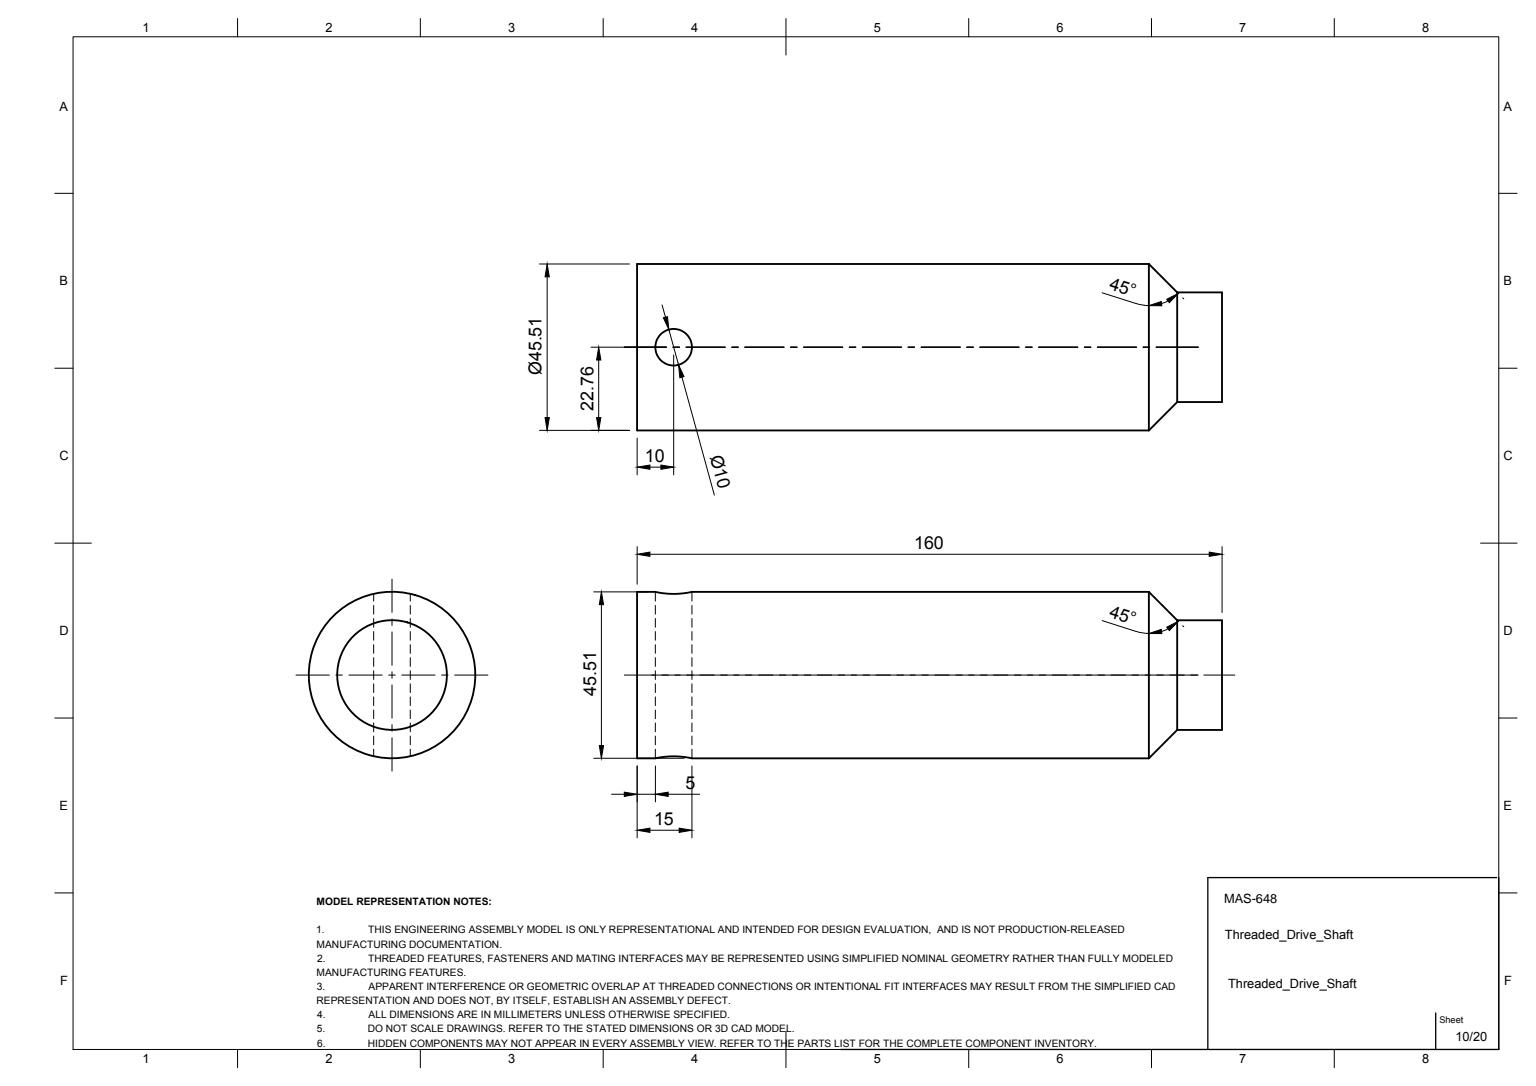
ISO-10303-21;
HEADER;
FILE_DESCRIPTION((''),'2;1');
FILE_NAME('Threaded_Drive_Shaft.step','2026-10-09T12:47:58-07:00',(''),(''),'','','');
FILE_SCHEMA (('AUTOMOTIVE_DESIGN { 1 0 10303 214 3 1 1 }'));
ENDSEC;
DATA;
#10=MECHANICAL_DESIGN_GEOMETRIC_PRESENTATION_REPRESENTATION('',(#313),#3475);
#31=CONICAL_SURFACE('',#2014,22.7551020408163,0.785398163397443) ;
#41=B_SPLINE_CURVE_WITH_KNOTS('',3,(#2969,#2970,#2971,#2972,#2973,#2974,
#2975,#2976,#2977,#2978,#2979,#2980,#2981,#2982,#2983,#2984,#2985,#2986,
#2987),.UNSPECIFIED.,.F.,.F.,(4,2,2,2,3,2,2,2,4),(-0.756034971359867,-0.567034005964369,
-0.378033040568871,-0.189016520284436,0.,0.189016520284436,0.378033040568871,
0.567034005964369,0.756034971359867),.UNSPECIFIED.) ;
#42=B_SPLINE_CURVE_WITH_KNOTS('',3,(#2989,#2990,#2991,#2992,#2993,#2994,
#2995,#2996,#2997,#2998),.UNSPECIFIED.,.F.,.F.,(4,2,2,2,4),(0.756034971359867,
0.945035936755365,1.13403690215086,1.3230534224353,1.51206994271973),
 .UNSPECIFIED.) ;
#43=B_SPLINE_CURVE_WITH_KNOTS('',3,(#3001,#3002,#3003,#3004,#3005,#3006,
#3007,#3008,#3009,#3010,#3011,#3012,#3013,#3014,#3015,#3016,#3017,#3018,
#3019,#3020,#3021,#3022,#3023,#3024,#3025,#3026,#3027,#3028,#3029,#3030,
#3031,#3032,#3033,#3034),.UNSPECIFIED.,.T.,.F.,(4,2,2,2,2,2,2,2,2,2,2,2,
2,2,2,2,4),(-3.02413988543947,-2.83512336515503,-2.6461068448706,-2.4571058794751,
-2.2681049140796,-2.0791039486841,-1.8901029832886,-1.70108646300417,-1.51206994271973,
-1.3230534224353,-1.13403690215086,-0.945035936755364,-0.756034971359867,
-0.567034005964369,-0.378033040568871,-0.189016520284436,0.),
 .UNSPECIFIED.) ;
#44=B_SPLINE_CURVE_WITH_KNOTS('',3,(#3035,#3036,#3037,#3038,#3039,#3040,
#3041,#3042,#3043,#3044),.UNSPECIFIED.,.F.,.F.,(4,2,2,2,4),(1.51206994271973,
1.70108646300417,1.8901029832886,2.0791039486841,2.2681049140796),
 .UNSPECIFIED.) ;
#147=FACE_BOUND('',#484,.T.) ;
#172=CIRCLE('',#2015,22.7551020408163) ;
#173=CIRCLE('',#2016,15.) ;
#174=CIRCLE('',#2018,22.7551020408163) ;
#175=CIRCLE('',#2020,15.) ;
#259=CYLINDRICAL_SURFACE('',#2013,5.00000000000002) ;
#260=CYLINDRICAL_SURFACE('',#2017,22.7551020408163) ;
#261=CYLINDRICAL_SURFACE('',#2019,15.) ;
#289=SHAPE_REPRESENTATION_RELATIONSHIP('SRR','None',#3544,#301) ;
#301=ADVANCED_BREP_SHAPE_REPRESENTATION('',(#325),#3464) ;
#313=STYLED_ITEM('',(#3628),#325) ;
#325=MANIFOLD_SOLID_BREP('Body1',#1827) ;
#361=FACE_OUTER_BOUND('',#481,.T.) ;
#362=FACE_OUTER_BOUND('',#482,.T.) ;
#363=FACE_OUTER_BOUND('',#483,.T.) ;
#364=FACE_OUTER_BOUND('',#485,.T.) ;
#365=FACE_OUTER_BOUND('',#486,.T.) ;
#366=FACE_OUTER_BOUND('',#487,.T.) ;
#481=EDGE_LOOP('',(#1320,#1321,#1322,#1323,#1324,#1325)) ;
#482=EDGE_LOOP('',(#1326,#1327,#1328,#1329)) ;
#483=EDGE_LOOP('',(#1330,#1331,#1332,#1333,#1334,#1335,#1336,#1337,#1338)) ;
#484=EDGE_LOOP('',(#1339)) ;
#485=EDGE_LOOP('',(#1340,#1341,#1342,#1343)) ;
#486=EDGE_LOOP('',(#1344)) ;
#487=EDGE_LOOP('',(#1345)) ;
#644=LINE('',#3000,#763) ;
#645=LINE('',#3049,#764) ;
#646=LINE('',#3054,#765) ;
#647=LINE('',#3055,#766) ;
#648=LINE('',#3058,#767) ;
#763=VECTOR('',#2361,5.00000000000002) ;
#764=VECTOR('',#2366,22.7551020408163) ;
#765=VECTOR('',#2373,22.7551020408163) ;
#766=VECTOR('',#2374,22.7551020408163) ;
#767=VECTOR('',#2377,15.) ;
#867=VERTEX_POINT('',#2967) ;
#868=VERTEX_POINT('',#2968) ;
#869=VERTEX_POINT('',#2988) ;
#870=VERTEX_POINT('',#2999) ;
#871=VERTEX_POINT('',#3046) ;
#872=VERTEX_POINT('',#3048) ;
#873=VERTEX_POINT('',#3052) ;
#874=VERTEX_POINT('',#3057) ;
#1032=EDGE_CURVE('',#867,#868,#41,.T.) ;
#1033=EDGE_CURVE('',#868,#869,#42,.T.) ;
#1034=EDGE_CURVE('',#869,#870,#644,.T.) ;
#1035=EDGE_CURVE('',#870,#870,#43,.T.) ;
#1036=EDGE_CURVE('',#869,#867,#44,.T.) ;
#1037=EDGE_CURVE('',#871,#871,#172,.T.) ;
#1038=EDGE_CURVE('',#871,#872,#645,.T.) ;
#1039=EDGE_CURVE('',#872,#872,#173,.T.) ;
#1040=EDGE_CURVE('',#873,#873,#174,.T.) ;
#1041=EDGE_CURVE('',#873,#867,#646,.T.) ;
#1042=EDGE_CURVE('',#868,#871,#647,.T.) ;
#1043=EDGE_CURVE('',#872,#874,#648,.T.) ;
#1044=EDGE_CURVE('',#874,#874,#175,.T.) ;
#1320=ORIENTED_EDGE('',*,*,#1032,.T.) ;
#1321=ORIENTED_EDGE('',*,*,#1033,.T.) ;
#1322=ORIENTED_EDGE('',*,*,#1034,.T.) ;
#1323=ORIENTED_EDGE('',*,*,#1035,.T.) ;
#1324=ORIENTED_EDGE('',*,*,#1034,.F.) ;
#1325=ORIENTED_EDGE('',*,*,#1036,.T.) ;
#1326=ORIENTED_EDGE('',*,*,#1037,.F.) ;
#1327=ORIENTED_EDGE('',*,*,#1038,.T.) ;
#1328=ORIENTED_EDGE('',*,*,#1039,.F.) ;
#1329=ORIENTED_EDGE('',*,*,#1038,.F.) ;
#1330=ORIENTED_EDGE('',*,*,#1040,.F.) ;
#1331=ORIENTED_EDGE('',*,*,#1041,.T.) ;
#1332=ORIENTED_EDGE('',*,*,#1036,.F.) ;
#1333=ORIENTED_EDGE('',*,*,#1033,.F.) ;
#1334=ORIENTED_EDGE('',*,*,#1042,.T.) ;
#1335=ORIENTED_EDGE('',*,*,#1037,.T.) ;
#1336=ORIENTED_EDGE('',*,*,#1042,.F.) ;
#1337=ORIENTED_EDGE('',*,*,#1032,.F.) ;
#1338=ORIENTED_EDGE('',*,*,#1041,.F.) ;
#1339=ORIENTED_EDGE('',*,*,#1035,.F.) ;
#1340=ORIENTED_EDGE('',*,*,#1039,.T.) ;
#1341=ORIENTED_EDGE('',*,*,#1043,.T.) ;
#1342=ORIENTED_EDGE('',*,*,#1044,.T.) ;
#1343=ORIENTED_EDGE('',*,*,#1043,.F.) ;
#1344=ORIENTED_EDGE('',*,*,#1044,.F.) ;
#1345=ORIENTED_EDGE('',*,*,#1040,.T.) ;
#1668=PLANE('',#2021) ;
#1669=PLANE('',#2022) ;
#1737=ADVANCED_FACE('',(#361),#259,.F.) ;
#1738=ADVANCED_FACE('',(#362),#31,.T.) ;
#1739=ADVANCED_FACE('',(#363,#147),#260,.T.) ;
#1740=ADVANCED_FACE('',(#364),#261,.T.) ;
#1741=ADVANCED_FACE('',(#365),#1668,.T.) ;
#1742=ADVANCED_FACE('',(#366),#1669,.T.) ;
#1827=CLOSED_SHELL('',(#1737,#1738,#1739,#1740,#1741,#1742)) ;
#2012=AXIS2_PLACEMENT_3D('',#2965,#2357,#2358) ;
#2013=AXIS2_PLACEMENT_3D('',#2966,#2359,#2360) ;
#2014=AXIS2_PLACEMENT_3D('',#3045,#2362,#2363) ;
#2015=AXIS2_PLACEMENT_3D('',#3047,#2364,#2365) ;
#2016=AXIS2_PLACEMENT_3D('',#3050,#2367,#2368) ;
#2017=AXIS2_PLACEMENT_3D('',#3051,#2369,#2370) ;
#2018=AXIS2_PLACEMENT_3D('',#3053,#2371,#2372) ;
#2019=AXIS2_PLACEMENT_3D('',#3056,#2375,#2376) ;
#2020=AXIS2_PLACEMENT_3D('',#3059,#2378,#2379) ;
#2021=AXIS2_PLACEMENT_3D('',#3060,#2380,#2381) ;
#2022=AXIS2_PLACEMENT_3D('',#3061,#2382,#2383) ;
#2357=DIRECTION('axis',(0.,0.,1.)) ;
#2358=DIRECTION('refdir',(1.,0.,0.)) ;
#2359=DIRECTION('center_axis',(0.,1.,0.)) ;
#2360=DIRECTION('ref_axis',(0.,0.,1.)) ;
#2361=DIRECTION('',(0.,1.,0.)) ;
#2362=DIRECTION('center_axis',(1.,2.84764536702765E-17,0.)) ;
#2363=DIRECTION('ref_axis',(-2.84764536702765E-17,1.,0.)) ;
#2364=DIRECTION('center_axis',(1.,2.84764536702765E-17,0.)) ;
#2365=DIRECTION('ref_axis',(2.84764536702765E-17,-1.,0.)) ;
#2366=DIRECTION('',(-0.707106781186551,0.707106781186544,8.65956056235489E-17)) ;
#2367=DIRECTION('center_axis',(-1.,-2.84764536702765E-17,0.)) ;
#2368=DIRECTION('ref_axis',(-2.84764536702765E-17,1.,0.)) ;
#2369=DIRECTION('center_axis',(1.,2.84764536702764E-17,0.)) ;
#2370=DIRECTION('ref_axis',(-2.84764536702764E-17,1.,0.)) ;
#2371=DIRECTION('center_axis',(1.,2.84764536702764E-17,0.)) ;
#2372=DIRECTION('ref_axis',(-2.84764536702764E-17,1.,0.)) ;
#2373=DIRECTION('',(-1.,-2.84764536702764E-17,0.)) ;
#2374=DIRECTION('',(-1.,-2.84764536702764E-17,0.)) ;
#2375=DIRECTION('center_axis',(1.,2.84764536702764E-17,0.)) ;
#2376=DIRECTION('ref_axis',(-2.84764536702764E-17,1.,0.)) ;
#2377=DIRECTION('',(-1.,-2.84764536702764E-17,0.)) ;
#2378=DIRECTION('center_axis',(1.,2.84764536702764E-17,0.)) ;
#2379=DIRECTION('ref_axis',(-2.84764536702764E-17,1.,0.)) ;
#2380=DIRECTION('center_axis',(-1.,-2.84764536702764E-17,0.)) ;
#2381=DIRECTION('ref_axis',(2.84764536702764E-17,-1.,0.)) ;
#2382=DIRECTION('center_axis',(1.,2.84764536702764E-17,0.)) ;
#2383=DIRECTION('ref_axis',(-2.84764536702764E-17,1.,0.)) ;
#2965=CARTESIAN_POINT('',(0.,0.,0.)) ;
#2966=CARTESIAN_POINT('Origin',(150.,-25.,0.)) ;
#2967=CARTESIAN_POINT('',(155.,-22.7551020408163,2.78562319867339E-15)) ;
#2968=CARTESIAN_POINT('',(145.,-22.7551020408163,-1.70559836960368E-15)) ;
#2969=CARTESIAN_POINT('Ctrl Pts',(155.,-22.7551020408163,2.77555756156289E-16)) ;
#2970=CARTESIAN_POINT('Ctrl Pts',(155.,-22.7551020408163,0.630003217984992)) ;
#2971=CARTESIAN_POINT('Ctrl Pts',(154.873673921497,-22.7263022754814,1.30061158958556)) ;
#2972=CARTESIAN_POINT('Ctrl Pts',(154.36275982174,-22.6222410731759,2.53191912872512)) ;
#2973=CARTESIAN_POINT('Ctrl Pts',(153.978283678305,-22.5483975458322,3.09278413356067)) ;
#2974=CARTESIAN_POINT('Ctrl Pts',(153.092747694998,-22.4091175126403,3.97832011686759)) ;
#2975=CARTESIAN_POINT('Ctrl Pts',(152.53189805439,-22.3344796638631,4.36276776282476)) ;
#2976=CARTESIAN_POINT('Ctrl Pts',(151.30064431178,-22.228588638716,4.87366114728546)) ;
#2977=CARTESIAN_POINT('Ctrl Pts',(150.630055067615,-22.19897900553,5.00000000000002)) ;
#2978=CARTESIAN_POINT('Ctrl Pts',(150.,-22.19897900553,5.00000000000002)) ;
#2979=CARTESIAN_POINT('Ctrl Pts',(149.369944932385,-22.19897900553,5.00000000000002)) ;
#2980=CARTESIAN_POINT('Ctrl Pts',(148.69935568822,-22.228588638716,4.87366114728546)) ;
#2981=CARTESIAN_POINT('Ctrl Pts',(147.46810194561,-22.3344796638631,4.36276776282476)) ;
#2982=CARTESIAN_POINT('Ctrl Pts',(146.907252305002,-22.4091175126403,3.97832011686759)) ;
#2983=CARTESIAN_POINT('Ctrl Pts',(146.021716321695,-22.5483975458322,3.09278413356067)) ;
#2984=CARTESIAN_POINT('Ctrl Pts',(145.63724017826,-22.6222410731759,2.53191912872511)) ;
#2985=CARTESIAN_POINT('Ctrl Pts',(145.126326078503,-22.7263022754814,1.30061158958555)) ;
#2986=CARTESIAN_POINT('Ctrl Pts',(145.,-22.7551020408163,0.630003217984992)) ;
#2987=CARTESIAN_POINT('Ctrl Pts',(145.,-22.7551020408163,-9.0205620750794E-16)) ;
#2988=CARTESIAN_POINT('',(150.,-22.19897900553,-5.00000000000002)) ;
#2989=CARTESIAN_POINT('Ctrl Pts',(145.,-22.7551020408163,-9.71445146547012E-16)) ;
#2990=CARTESIAN_POINT('Ctrl Pts',(145.,-22.7551020408163,-0.630003217984994)) ;
#2991=CARTESIAN_POINT('Ctrl Pts',(145.126326078503,-22.7263022754814,-1.30061158958556)) ;
#2992=CARTESIAN_POINT('Ctrl Pts',(145.63724017826,-22.6222410731759,-2.53191912872513)) ;
#2993=CARTESIAN_POINT('Ctrl Pts',(146.021716321695,-22.5483975458322,-3.09278413356067)) ;
#2994=CARTESIAN_POINT('Ctrl Pts',(146.907252305002,-22.4091175126403,-3.97832011686759)) ;
#2995=CARTESIAN_POINT('Ctrl Pts',(147.46810194561,-22.3344796638631,-4.36276776282476)) ;
#2996=CARTESIAN_POINT('Ctrl Pts',(148.69935568822,-22.228588638716,-4.87366114728546)) ;
#2997=CARTESIAN_POINT('Ctrl Pts',(149.369944932385,-22.19897900553,-5.00000000000002)) ;
#2998=CARTESIAN_POINT('Ctrl Pts',(150.,-22.19897900553,-5.00000000000002)) ;
#2999=CARTESIAN_POINT('',(150.,22.19897900553,-5.00000000000002)) ;
#3000=CARTESIAN_POINT('',(150.,-25.,-5.00000000000002)) ;
#3001=CARTESIAN_POINT('Ctrl Pts',(150.,22.19897900553,5.00000000000002)) ;
#3002=CARTESIAN_POINT('Ctrl Pts',(150.630055067615,22.19897900553,5.00000000000002)) ;
#3003=CARTESIAN_POINT('Ctrl Pts',(151.30064431178,22.228588638716,4.87366114728546)) ;
#3004=CARTESIAN_POINT('Ctrl Pts',(152.53189805439,22.3344796638632,4.36276776282476)) ;
#3005=CARTESIAN_POINT('Ctrl Pts',(153.092747694998,22.4091175126403,3.97832011686759)) ;
#3006=CARTESIAN_POINT('Ctrl Pts',(153.978283678305,22.5483975458322,3.09278413356067)) ;
#3007=CARTESIAN_POINT('Ctrl Pts',(154.36275982174,22.6222410731759,2.53191912872511)) ;
#3008=CARTESIAN_POINT('Ctrl Pts',(154.873673921497,22.7263022754814,1.30061158958554)) ;
#3009=CARTESIAN_POINT('Ctrl Pts',(155.,22.7551020408163,0.630003217984991)) ;
#3010=CARTESIAN_POINT('Ctrl Pts',(155.,22.7551020408163,-0.630003217984991)) ;
#3011=CARTESIAN_POINT('Ctrl Pts',(154.873673921497,22.7263022754814,-1.30061158958554)) ;
#3012=CARTESIAN_POINT('Ctrl Pts',(154.36275982174,22.6222410731759,-2.5319191287251)) ;
#3013=CARTESIAN_POINT('Ctrl Pts',(153.978283678305,22.5483975458322,-3.09278413356067)) ;
#3014=CARTESIAN_POINT('Ctrl Pts',(153.092747694998,22.4091175126403,-3.97832011686758)) ;
#3015=CARTESIAN_POINT('Ctrl Pts',(152.53189805439,22.3344796638632,-4.36276776282476)) ;
#3016=CARTESIAN_POINT('Ctrl Pts',(151.30064431178,22.228588638716,-4.87366114728546)) ;
#3017=CARTESIAN_POINT('Ctrl Pts',(150.630055067615,22.19897900553,-5.00000000000002)) ;
#3018=CARTESIAN_POINT('Ctrl Pts',(149.369944932385,22.19897900553,-5.00000000000002)) ;
#3019=CARTESIAN_POINT('Ctrl Pts',(148.69935568822,22.228588638716,-4.87366114728546)) ;
#3020=CARTESIAN_POINT('Ctrl Pts',(147.46810194561,22.3344796638631,-4.36276776282476)) ;
#3021=CARTESIAN_POINT('Ctrl Pts',(146.907252305002,22.4091175126403,-3.97832011686759)) ;
#3022=CARTESIAN_POINT('Ctrl Pts',(146.021716321695,22.5483975458322,-3.09278413356067)) ;
#3023=CARTESIAN_POINT('Ctrl Pts',(145.63724017826,22.6222410731759,-2.53191912872511)) ;
#3024=CARTESIAN_POINT('Ctrl Pts',(145.126326078503,22.7263022754814,-1.30061158958555)) ;
#3025=CARTESIAN_POINT('Ctrl Pts',(145.,22.7551020408163,-0.630003217984993)) ;
#3026=CARTESIAN_POINT('Ctrl Pts',(145.,22.7551020408163,0.630003217984992)) ;
#3027=CARTESIAN_POINT('Ctrl Pts',(145.126326078503,22.7263022754814,1.30061158958556)) ;
#3028=CARTESIAN_POINT('Ctrl Pts',(145.63724017826,22.6222410731759,2.53191912872512)) ;
#3029=CARTESIAN_POINT('Ctrl Pts',(146.021716321695,22.5483975458322,3.09278413356067)) ;
#3030=CARTESIAN_POINT('Ctrl Pts',(146.907252305002,22.4091175126403,3.97832011686759)) ;
#3031=CARTESIAN_POINT('Ctrl Pts',(147.46810194561,22.3344796638632,4.36276776282476)) ;
#3032=CARTESIAN_POINT('Ctrl Pts',(148.69935568822,22.228588638716,4.87366114728546)) ;
#3033=CARTESIAN_POINT('Ctrl Pts',(149.369944932385,22.19897900553,5.00000000000002)) ;
#3034=CARTESIAN_POINT('Ctrl Pts',(150.,22.19897900553,5.00000000000002)) ;
#3035=CARTESIAN_POINT('Ctrl Pts',(150.,-22.19897900553,-5.00000000000002)) ;
#3036=CARTESIAN_POINT('Ctrl Pts',(150.630055067615,-22.19897900553,-5.00000000000002)) ;
#3037=CARTESIAN_POINT('Ctrl Pts',(151.30064431178,-22.228588638716,-4.87366114728547)) ;
#3038=CARTESIAN_POINT('Ctrl Pts',(152.53189805439,-22.3344796638631,-4.36276776282477)) ;
#3039=CARTESIAN_POINT('Ctrl Pts',(153.092747694998,-22.4091175126403,-3.97832011686758)) ;
#3040=CARTESIAN_POINT('Ctrl Pts',(153.978283678305,-22.5483975458322,-3.09278413356067)) ;
#3041=CARTESIAN_POINT('Ctrl Pts',(154.36275982174,-22.6222410731759,-2.53191912872511)) ;
#3042=CARTESIAN_POINT('Ctrl Pts',(154.873673921497,-22.7263022754814,-1.30061158958555)) ;
#3043=CARTESIAN_POINT('Ctrl Pts',(155.,-22.7551020408163,-0.630003217984992)) ;
#3044=CARTESIAN_POINT('Ctrl Pts',(155.,-22.7551020408163,0.)) ;
#3045=CARTESIAN_POINT('Origin',(20.0000000000002,5.69529073405534E-16,0.)) ;
#3046=CARTESIAN_POINT('',(20.0000000000002,-22.7551020408163,-2.78669628785571E-15)) ;
#3047=CARTESIAN_POINT('Origin',(20.0000000000002,5.69529073405534E-16,0.)) ;
#3048=CARTESIAN_POINT('',(12.2448979591838,-15.,-1.83697019872103E-15)) ;
#3049=CARTESIAN_POINT('',(20.0000000000002,-22.7551020408163,-2.78669628785571E-15)) ;
#3050=CARTESIAN_POINT('Origin',(12.2448979591838,3.48691269431959E-16,0.)) ;
#3051=CARTESIAN_POINT('Origin',(160.,4.55623258724423E-15,0.)) ;
#3052=CARTESIAN_POINT('',(160.,-22.7551020408163,-2.78669628785571E-15)) ;
#3053=CARTESIAN_POINT('Origin',(160.,4.55623258724423E-15,0.)) ;
#3054=CARTESIAN_POINT('',(160.,-22.7551020408163,-2.78669628785571E-15)) ;
#3055=CARTESIAN_POINT('',(160.,-22.7551020408163,-2.78669628785571E-15)) ;
#3056=CARTESIAN_POINT('Origin',(160.,4.55623258724423E-15,0.)) ;
#3057=CARTESIAN_POINT('',(0.,-15.,-1.83697019872103E-15)) ;
#3058=CARTESIAN_POINT('',(160.,-15.,-1.83697019872103E-15)) ;
#3059=CARTESIAN_POINT('Origin',(0.,0.,0.)) ;
#3060=CARTESIAN_POINT('Origin',(2.13573402527073E-16,6.08181310226549E-33,
0.)) ;
#3061=CARTESIAN_POINT('Origin',(160.,22.7551020408163,0.)) ;
#3446=UNCERTAINTY_MEASURE_WITH_UNIT(LENGTH_MEASURE(0.01),#3476,
'DISTANCE_ACCURACY_VALUE',
'Maximum model space distance between geometric entities at asserted c
onnectivities') ;
#3457=UNCERTAINTY_MEASURE_WITH_UNIT(LENGTH_MEASURE(0.01),#3476,
'DISTANCE_ACCURACY_VALUE',
'Maximum model space distance between geometric entities at asserted c
onnectivities') ;
#3464=(
GEOMETRIC_REPRESENTATION_CONTEXT(3)
GLOBAL_UNCERTAINTY_ASSIGNED_CONTEXT((#3446))
GLOBAL_UNIT_ASSIGNED_CONTEXT((#3476,#3478,#3479))
REPRESENTATION_CONTEXT('','3D')
) ;
#3475=(
GEOMETRIC_REPRESENTATION_CONTEXT(3)
GLOBAL_UNCERTAINTY_ASSIGNED_CONTEXT((#3457))
GLOBAL_UNIT_ASSIGNED_CONTEXT((#3476,#3478,#3479))
REPRESENTATION_CONTEXT('','3D')
) ;
#3476=(
LENGTH_UNIT()
NAMED_UNIT(*)
SI_UNIT(.MILLI.,.METRE.)
) ;
#3478=(
NAMED_UNIT(*)
PLANE_ANGLE_UNIT()
SI_UNIT($,.RADIAN.)
) ;
#3479=(
NAMED_UNIT(*)
SI_UNIT($,.STERADIAN.)
SOLID_ANGLE_UNIT()
) ;
#3486=SHAPE_DEFINITION_REPRESENTATION(#3507,#3544) ;
#3507=PRODUCT_DEFINITION_SHAPE('',$,#3562) ;
#3544=SHAPE_REPRESENTATION('',(#2012),#3464) ;
#3555=PRODUCT_DEFINITION_CONTEXT('part definition',#3608,'design') ;
#3562=PRODUCT_DEFINITION('Threaded_Drive_Shaft','Threaded_Drive_Shaft',#3579,#3555) ;
#3579=PRODUCT_DEFINITION_FORMATION('',$,#3616) ;
#3608=APPLICATION_CONTEXT(
'Core Data for Automotive Mechanical Design Process') ;
#3609=PRODUCT_CONTEXT('part definition',#3608,'mechanical') ;
#3616=PRODUCT('Threaded_Drive_Shaft','Threaded_Drive_Shaft',$,(#3609)) ;
#3628=PRESENTATION_STYLE_ASSIGNMENT((#3630)) ;
#3630=SURFACE_STYLE_USAGE(.BOTH.,#3632) ;
#3632=SURFACE_SIDE_STYLE('',(#3634)) ;
#3634=SURFACE_STYLE_FILL_AREA(#3636) ;
#3636=FILL_AREA_STYLE('Opaque(202,209,238)',(#3638)) ;
#3638=FILL_AREA_STYLE_COLOUR('Opaque(202,209,238)',#3640) ;
#3640=COLOUR_RGB('Opaque(202,209,238)', 0.09019608, 0.27058824, 0.51372549) ;
ENDSEC;
END-ISO-10303-21;
